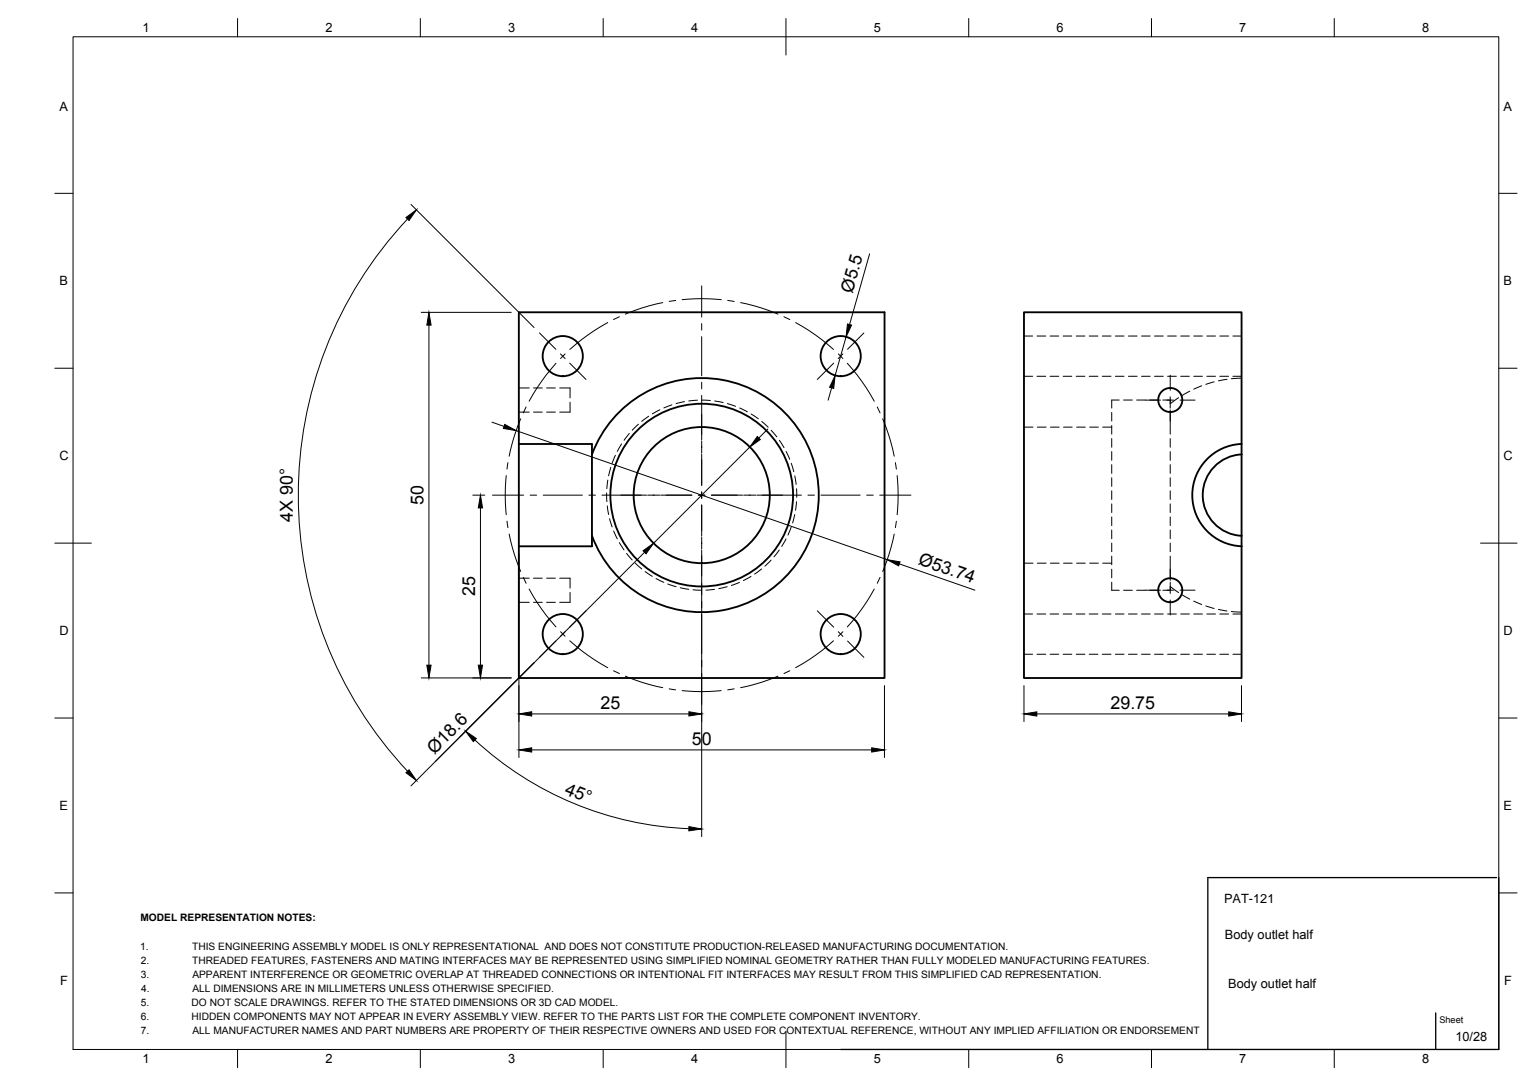
ISO-10303-21;
HEADER;
/* Generated by software containing ST-Developer
 * from STEP Tools, Inc. (www.steptools.com) 
 */

FILE_DESCRIPTION(
/* description */ ('Wall-mounted air drop station'),
/* implementation_level */ '2;1');

FILE_NAME(
/* name */ 'Body outlet half.step',
/* time_stamp */ '2026-10-28T22:16:19-07:00',
/* author */ (''),
/* organization */ (''),
/* preprocessor_version */ 'ST-DEVELOPER v20.2',
/* originating_system */ 'Autodesk Translation Framework v15.17.0.0',
/* authorisation */ '');

FILE_SCHEMA (('AUTOMOTIVE_DESIGN { 1 0 10303 214 3 1 1 }'));
ENDSEC;

DATA;
#10=MECHANICAL_DESIGN_GEOMETRIC_PRESENTATION_REPRESENTATION('',(#350),#10517);
#259=SPHERICAL_SURFACE('',#6460,1.6);
#292=SHAPE_REPRESENTATION_RELATIONSHIP('SRR','None',#10649,#321);
#321=ADVANCED_BREP_SHAPE_REPRESENTATION('',(#379),#10493);
#350=STYLED_ITEM('',(#10853),#379);
#379=MANIFOLD_SOLID_BREP('Body1',#5889);
#449=FACE_BOUND('',#1275,.T.);
#450=FACE_BOUND('',#1276,.T.);
#451=FACE_BOUND('',#1280,.T.);
#452=FACE_BOUND('',#1282,.T.);
#453=FACE_BOUND('',#1284,.T.);
#454=FACE_BOUND('',#1286,.T.);
#455=FACE_BOUND('',#1287,.T.);
#456=FACE_BOUND('',#1288,.T.);
#457=FACE_BOUND('',#1289,.T.);
#458=FACE_BOUND('',#1290,.T.);
#459=FACE_BOUND('',#1293,.T.);
#460=FACE_BOUND('',#1294,.T.);
#461=FACE_BOUND('',#1295,.T.);
#462=FACE_BOUND('',#1296,.T.);
#591=PLANE('',#6428);
#592=PLANE('',#6432);
#593=PLANE('',#6448);
#594=PLANE('',#6450);
#595=PLANE('',#6457);
#596=PLANE('',#6458);
#597=PLANE('',#6462);
#598=PLANE('',#6463);
#599=PLANE('',#6464);
#600=PLANE('',#6465);
#601=PLANE('',#6466);
#859=FACE_OUTER_BOUND('',#1264,.T.);
#860=FACE_OUTER_BOUND('',#1265,.T.);
#861=FACE_OUTER_BOUND('',#1266,.T.);
#862=FACE_OUTER_BOUND('',#1267,.T.);
#863=FACE_OUTER_BOUND('',#1268,.T.);
#864=FACE_OUTER_BOUND('',#1269,.T.);
#865=FACE_OUTER_BOUND('',#1270,.T.);
#866=FACE_OUTER_BOUND('',#1271,.T.);
#867=FACE_OUTER_BOUND('',#1272,.T.);
#868=FACE_OUTER_BOUND('',#1273,.T.);
#869=FACE_OUTER_BOUND('',#1274,.T.);
#870=FACE_OUTER_BOUND('',#1277,.T.);
#871=FACE_OUTER_BOUND('',#1278,.T.);
#872=FACE_OUTER_BOUND('',#1279,.T.);
#873=FACE_OUTER_BOUND('',#1281,.T.);
#874=FACE_OUTER_BOUND('',#1283,.T.);
#875=FACE_OUTER_BOUND('',#1285,.T.);
#876=FACE_OUTER_BOUND('',#1291,.T.);
#877=FACE_OUTER_BOUND('',#1292,.T.);
#878=FACE_OUTER_BOUND('',#1297,.T.);
#879=FACE_OUTER_BOUND('',#1298,.T.);
#1264=EDGE_LOOP('',(#4415,#4416,#4417,#4418));
#1265=EDGE_LOOP('',(#4419));
#1266=EDGE_LOOP('',(#4420,#4421,#4422,#4423));
#1267=EDGE_LOOP('',(#4424));
#1268=EDGE_LOOP('',(#4425,#4426,#4427,#4428));
#1269=EDGE_LOOP('',(#4429,#4430,#4431,#4432));
#1270=EDGE_LOOP('',(#4433,#4434,#4435,#4436));
#1271=EDGE_LOOP('',(#4437,#4438,#4439,#4440));
#1272=EDGE_LOOP('',(#4441,#4442,#4443,#4444));
#1273=EDGE_LOOP('',(#4445,#4446,#4447,#4448));
#1274=EDGE_LOOP('',(#4449,#4450,#4451,#4452,#4453,#4454));
#1275=EDGE_LOOP('',(#4455));
#1276=EDGE_LOOP('',(#4456));
#1277=EDGE_LOOP('',(#4457,#4458,#4459,#4460));
#1278=EDGE_LOOP('',(#4461,#4462,#4463,#4464));
#1279=EDGE_LOOP('',(#4465));
#1280=EDGE_LOOP('',(#4466));
#1281=EDGE_LOOP('',(#4467));
#1282=EDGE_LOOP('',(#4468));
#1283=EDGE_LOOP('',(#4469,#4470));
#1284=EDGE_LOOP('',(#4471));
#1285=EDGE_LOOP('',(#4472,#4473,#4474,#4475));
#1286=EDGE_LOOP('',(#4476));
#1287=EDGE_LOOP('',(#4477));
#1288=EDGE_LOOP('',(#4478));
#1289=EDGE_LOOP('',(#4479));
#1290=EDGE_LOOP('',(#4480));
#1291=EDGE_LOOP('',(#4481,#4482,#4483,#4484));
#1292=EDGE_LOOP('',(#4485,#4486,#4487,#4488,#4489,#4490,#4491,#4492,#4493,
#4494));
#1293=EDGE_LOOP('',(#4495));
#1294=EDGE_LOOP('',(#4496));
#1295=EDGE_LOOP('',(#4497));
#1296=EDGE_LOOP('',(#4498));
#1297=EDGE_LOOP('',(#4499,#4500,#4501,#4502));
#1298=EDGE_LOOP('',(#4503,#4504,#4505,#4506));
#1736=LINE('',#9251,#2200);
#1737=LINE('',#9258,#2201);
#1738=LINE('',#9265,#2202);
#1739=LINE('',#9271,#2203);
#1740=LINE('',#9277,#2204);
#1741=LINE('',#9283,#2205);
#1742=LINE('',#9288,#2206);
#1743=LINE('',#9292,#2207);
#1744=LINE('',#9296,#2208);
#1745=LINE('',#9299,#2209);
#1746=LINE('',#9302,#2210);
#1747=LINE('',#9304,#2211);
#1748=LINE('',#9306,#2212);
#1749=LINE('',#9308,#2213);
#1750=LINE('',#9309,#2214);
#1751=LINE('',#9314,#2215);
#1752=LINE('',#9320,#2216);
#1753=LINE('',#9331,#2217);
#1754=LINE('',#9332,#2218);
#1755=LINE('',#9333,#2219);
#1756=LINE('',#9336,#2220);
#1757=LINE('',#9337,#2221);
#1758=LINE('',#9340,#2222);
#1759=LINE('',#9341,#2223);
#1760=LINE('',#9343,#2224);
#2200=VECTOR('',#7452,0.165);
#2201=VECTOR('',#7461,0.165);
#2202=VECTOR('',#7470,0.275);
#2203=VECTOR('',#7477,0.275);
#2204=VECTOR('',#7484,0.275);
#2205=VECTOR('',#7491,0.275);
#2206=VECTOR('',#7496,1.);
#2207=VECTOR('',#7499,1.);
#2208=VECTOR('',#7504,1.);
#2209=VECTOR('',#7507,1.);
#2210=VECTOR('',#7510,1.);
#2211=VECTOR('',#7511,1.);
#2212=VECTOR('',#7512,1.);
#2213=VECTOR('',#7513,1.);
#2214=VECTOR('',#7514,1.);
#2215=VECTOR('',#7519,0.93);
#2216=VECTOR('',#7526,1.3);
#2217=VECTOR('',#7541,1.);
#2218=VECTOR('',#7542,1.);
#2219=VECTOR('',#7543,1.);
#2220=VECTOR('',#7546,1.);
#2221=VECTOR('',#7547,1.);
#2222=VECTOR('',#7550,1.);
#2223=VECTOR('',#7551,1.);
#2224=VECTOR('',#7554,1.);
#2597=CIRCLE('',#6426,0.165);
#2598=CIRCLE('',#6427,0.165);
#2599=CIRCLE('',#6430,0.165);
#2600=CIRCLE('',#6431,0.165);
#2601=CIRCLE('',#6434,0.275);
#2602=CIRCLE('',#6435,0.275);
#2603=CIRCLE('',#6437,0.275);
#2604=CIRCLE('',#6438,0.275);
#2605=CIRCLE('',#6440,0.275);
#2606=CIRCLE('',#6441,0.275);
#2607=CIRCLE('',#6443,0.275);
#2608=CIRCLE('',#6444,0.275);
#2609=CIRCLE('',#6446,0.7);
#2610=CIRCLE('',#6447,0.7);
#2611=CIRCLE('',#6449,0.556776436283003);
#2612=CIRCLE('',#6452,0.93);
#2613=CIRCLE('',#6453,0.93);
#2614=CIRCLE('',#6455,1.3);
#2615=CIRCLE('',#6456,1.3);
#2616=CIRCLE('',#6459,1.24899959967968);
#2617=CIRCLE('',#6461,1.59980467557762);
#2912=VERTEX_POINT('',#9248);
#2913=VERTEX_POINT('',#9250);
#2914=VERTEX_POINT('',#9255);
#2915=VERTEX_POINT('',#9257);
#2916=VERTEX_POINT('',#9262);
#2917=VERTEX_POINT('',#9264);
#2918=VERTEX_POINT('',#9268);
#2919=VERTEX_POINT('',#9270);
#2920=VERTEX_POINT('',#9274);
#2921=VERTEX_POINT('',#9276);
#2922=VERTEX_POINT('',#9280);
#2923=VERTEX_POINT('',#9282);
#2924=VERTEX_POINT('',#9286);
#2925=VERTEX_POINT('',#9287);
#2926=VERTEX_POINT('',#9289);
#2927=VERTEX_POINT('',#9291);
#2928=VERTEX_POINT('',#9295);
#2929=VERTEX_POINT('',#9297);
#2930=VERTEX_POINT('',#9301);
#2931=VERTEX_POINT('',#9303);
#2932=VERTEX_POINT('',#9305);
#2933=VERTEX_POINT('',#9307);
#2934=VERTEX_POINT('',#9311);
#2935=VERTEX_POINT('',#9313);
#2936=VERTEX_POINT('',#9317);
#2937=VERTEX_POINT('',#9319);
#2938=VERTEX_POINT('',#9324);
#2939=VERTEX_POINT('',#9329);
#2940=VERTEX_POINT('',#9330);
#2941=VERTEX_POINT('',#9335);
#2942=VERTEX_POINT('',#9339);
#3465=EDGE_CURVE('',#2912,#2912,#2597,.T.);
#3466=EDGE_CURVE('',#2912,#2913,#1736,.T.);
#3467=EDGE_CURVE('',#2913,#2913,#2598,.T.);
#3468=EDGE_CURVE('',#2914,#2914,#2599,.T.);
#3469=EDGE_CURVE('',#2914,#2915,#1737,.T.);
#3470=EDGE_CURVE('',#2915,#2915,#2600,.T.);
#3471=EDGE_CURVE('',#2916,#2916,#2601,.T.);
#3472=EDGE_CURVE('',#2916,#2917,#1738,.T.);
#3473=EDGE_CURVE('',#2917,#2917,#2602,.T.);
#3474=EDGE_CURVE('',#2918,#2918,#2603,.T.);
#3475=EDGE_CURVE('',#2918,#2919,#1739,.T.);
#3476=EDGE_CURVE('',#2919,#2919,#2604,.T.);
#3477=EDGE_CURVE('',#2920,#2920,#2605,.T.);
#3478=EDGE_CURVE('',#2920,#2921,#1740,.T.);
#3479=EDGE_CURVE('',#2921,#2921,#2606,.T.);
#3480=EDGE_CURVE('',#2922,#2922,#2607,.T.);
#3481=EDGE_CURVE('',#2922,#2923,#1741,.T.);
#3482=EDGE_CURVE('',#2923,#2923,#2608,.T.);
#3483=EDGE_CURVE('',#2924,#2925,#1742,.T.);
#3484=EDGE_CURVE('',#2926,#2924,#2609,.T.);
#3485=EDGE_CURVE('',#2927,#2926,#1743,.T.);
#3486=EDGE_CURVE('',#2925,#2927,#2610,.T.);
#3487=EDGE_CURVE('',#2928,#2924,#1744,.T.);
#3488=EDGE_CURVE('',#2929,#2928,#2611,.T.);
#3489=EDGE_CURVE('',#2926,#2929,#1745,.T.);
#3490=EDGE_CURVE('',#2927,#2930,#1746,.T.);
#3491=EDGE_CURVE('',#2930,#2931,#1747,.T.);
#3492=EDGE_CURVE('',#2931,#2932,#1748,.T.);
#3493=EDGE_CURVE('',#2932,#2933,#1749,.T.);
#3494=EDGE_CURVE('',#2933,#2925,#1750,.T.);
#3495=EDGE_CURVE('',#2934,#2934,#2612,.T.);
#3496=EDGE_CURVE('',#2934,#2935,#1751,.T.);
#3497=EDGE_CURVE('',#2935,#2935,#2613,.T.);
#3498=EDGE_CURVE('',#2936,#2936,#2614,.T.);
#3499=EDGE_CURVE('',#2936,#2937,#1752,.T.);
#3500=EDGE_CURVE('',#2937,#2937,#2615,.T.);
#3501=EDGE_CURVE('',#2938,#2938,#2616,.T.);
#3502=EDGE_CURVE('',#2929,#2928,#2617,.T.);
#3503=EDGE_CURVE('',#2939,#2940,#1753,.T.);
#3504=EDGE_CURVE('',#2940,#2932,#1754,.T.);
#3505=EDGE_CURVE('',#2939,#2931,#1755,.T.);
#3506=EDGE_CURVE('',#2941,#2939,#1756,.T.);
#3507=EDGE_CURVE('',#2941,#2930,#1757,.T.);
#3508=EDGE_CURVE('',#2942,#2933,#1758,.T.);
#3509=EDGE_CURVE('',#2942,#2941,#1759,.T.);
#3510=EDGE_CURVE('',#2940,#2942,#1760,.T.);
#4415=ORIENTED_EDGE('',*,*,#3465,.F.);
#4416=ORIENTED_EDGE('',*,*,#3466,.T.);
#4417=ORIENTED_EDGE('',*,*,#3467,.F.);
#4418=ORIENTED_EDGE('',*,*,#3466,.F.);
#4419=ORIENTED_EDGE('',*,*,#3465,.T.);
#4420=ORIENTED_EDGE('',*,*,#3468,.F.);
#4421=ORIENTED_EDGE('',*,*,#3469,.T.);
#4422=ORIENTED_EDGE('',*,*,#3470,.F.);
#4423=ORIENTED_EDGE('',*,*,#3469,.F.);
#4424=ORIENTED_EDGE('',*,*,#3468,.T.);
#4425=ORIENTED_EDGE('',*,*,#3471,.F.);
#4426=ORIENTED_EDGE('',*,*,#3472,.T.);
#4427=ORIENTED_EDGE('',*,*,#3473,.F.);
#4428=ORIENTED_EDGE('',*,*,#3472,.F.);
#4429=ORIENTED_EDGE('',*,*,#3474,.F.);
#4430=ORIENTED_EDGE('',*,*,#3475,.T.);
#4431=ORIENTED_EDGE('',*,*,#3476,.F.);
#4432=ORIENTED_EDGE('',*,*,#3475,.F.);
#4433=ORIENTED_EDGE('',*,*,#3477,.F.);
#4434=ORIENTED_EDGE('',*,*,#3478,.T.);
#4435=ORIENTED_EDGE('',*,*,#3479,.F.);
#4436=ORIENTED_EDGE('',*,*,#3478,.F.);
#4437=ORIENTED_EDGE('',*,*,#3480,.F.);
#4438=ORIENTED_EDGE('',*,*,#3481,.T.);
#4439=ORIENTED_EDGE('',*,*,#3482,.F.);
#4440=ORIENTED_EDGE('',*,*,#3481,.F.);
#4441=ORIENTED_EDGE('',*,*,#3483,.F.);
#4442=ORIENTED_EDGE('',*,*,#3484,.F.);
#4443=ORIENTED_EDGE('',*,*,#3485,.F.);
#4444=ORIENTED_EDGE('',*,*,#3486,.F.);
#4445=ORIENTED_EDGE('',*,*,#3487,.F.);
#4446=ORIENTED_EDGE('',*,*,#3488,.F.);
#4447=ORIENTED_EDGE('',*,*,#3489,.F.);
#4448=ORIENTED_EDGE('',*,*,#3484,.T.);
#4449=ORIENTED_EDGE('',*,*,#3486,.T.);
#4450=ORIENTED_EDGE('',*,*,#3490,.T.);
#4451=ORIENTED_EDGE('',*,*,#3491,.T.);
#4452=ORIENTED_EDGE('',*,*,#3492,.T.);
#4453=ORIENTED_EDGE('',*,*,#3493,.T.);
#4454=ORIENTED_EDGE('',*,*,#3494,.T.);
#4455=ORIENTED_EDGE('',*,*,#3467,.T.);
#4456=ORIENTED_EDGE('',*,*,#3470,.T.);
#4457=ORIENTED_EDGE('',*,*,#3495,.F.);
#4458=ORIENTED_EDGE('',*,*,#3496,.T.);
#4459=ORIENTED_EDGE('',*,*,#3497,.F.);
#4460=ORIENTED_EDGE('',*,*,#3496,.F.);
#4461=ORIENTED_EDGE('',*,*,#3498,.F.);
#4462=ORIENTED_EDGE('',*,*,#3499,.T.);
#4463=ORIENTED_EDGE('',*,*,#3500,.T.);
#4464=ORIENTED_EDGE('',*,*,#3499,.F.);
#4465=ORIENTED_EDGE('',*,*,#3500,.F.);
#4466=ORIENTED_EDGE('',*,*,#3495,.T.);
#4467=ORIENTED_EDGE('',*,*,#3498,.T.);
#4468=ORIENTED_EDGE('',*,*,#3501,.F.);
#4469=ORIENTED_EDGE('',*,*,#3488,.T.);
#4470=ORIENTED_EDGE('',*,*,#3502,.F.);
#4471=ORIENTED_EDGE('',*,*,#3501,.T.);
#4472=ORIENTED_EDGE('',*,*,#3503,.T.);
#4473=ORIENTED_EDGE('',*,*,#3504,.T.);
#4474=ORIENTED_EDGE('',*,*,#3492,.F.);
#4475=ORIENTED_EDGE('',*,*,#3505,.F.);
#4476=ORIENTED_EDGE('',*,*,#3497,.T.);
#4477=ORIENTED_EDGE('',*,*,#3482,.T.);
#4478=ORIENTED_EDGE('',*,*,#3479,.T.);
#4479=ORIENTED_EDGE('',*,*,#3476,.T.);
#4480=ORIENTED_EDGE('',*,*,#3473,.T.);
#4481=ORIENTED_EDGE('',*,*,#3506,.T.);
#4482=ORIENTED_EDGE('',*,*,#3505,.T.);
#4483=ORIENTED_EDGE('',*,*,#3491,.F.);
#4484=ORIENTED_EDGE('',*,*,#3507,.F.);
#4485=ORIENTED_EDGE('',*,*,#3483,.T.);
#4486=ORIENTED_EDGE('',*,*,#3494,.F.);
#4487=ORIENTED_EDGE('',*,*,#3508,.F.);
#4488=ORIENTED_EDGE('',*,*,#3509,.T.);
#4489=ORIENTED_EDGE('',*,*,#3507,.T.);
#4490=ORIENTED_EDGE('',*,*,#3490,.F.);
#4491=ORIENTED_EDGE('',*,*,#3485,.T.);
#4492=ORIENTED_EDGE('',*,*,#3489,.T.);
#4493=ORIENTED_EDGE('',*,*,#3502,.T.);
#4494=ORIENTED_EDGE('',*,*,#3487,.T.);
#4495=ORIENTED_EDGE('',*,*,#3471,.T.);
#4496=ORIENTED_EDGE('',*,*,#3474,.T.);
#4497=ORIENTED_EDGE('',*,*,#3477,.T.);
#4498=ORIENTED_EDGE('',*,*,#3480,.T.);
#4499=ORIENTED_EDGE('',*,*,#3510,.T.);
#4500=ORIENTED_EDGE('',*,*,#3508,.T.);
#4501=ORIENTED_EDGE('',*,*,#3493,.F.);
#4502=ORIENTED_EDGE('',*,*,#3504,.F.);
#4503=ORIENTED_EDGE('',*,*,#3510,.F.);
#4504=ORIENTED_EDGE('',*,*,#3503,.F.);
#4505=ORIENTED_EDGE('',*,*,#3506,.F.);
#4506=ORIENTED_EDGE('',*,*,#3509,.F.);
#5466=CYLINDRICAL_SURFACE('',#6425,0.165);
#5467=CYLINDRICAL_SURFACE('',#6429,0.165);
#5468=CYLINDRICAL_SURFACE('',#6433,0.275);
#5469=CYLINDRICAL_SURFACE('',#6436,0.275);
#5470=CYLINDRICAL_SURFACE('',#6439,0.275);
#5471=CYLINDRICAL_SURFACE('',#6442,0.275);
#5472=CYLINDRICAL_SURFACE('',#6445,0.7);
#5473=CYLINDRICAL_SURFACE('',#6451,0.93);
#5474=CYLINDRICAL_SURFACE('',#6454,1.3);
#5632=ADVANCED_FACE('',(#859),#5466,.F.);
#5633=ADVANCED_FACE('',(#860),#591,.T.);
#5634=ADVANCED_FACE('',(#861),#5467,.F.);
#5635=ADVANCED_FACE('',(#862),#592,.T.);
#5636=ADVANCED_FACE('',(#863),#5468,.F.);
#5637=ADVANCED_FACE('',(#864),#5469,.F.);
#5638=ADVANCED_FACE('',(#865),#5470,.F.);
#5639=ADVANCED_FACE('',(#866),#5471,.F.);
#5640=ADVANCED_FACE('',(#867),#5472,.F.);
#5641=ADVANCED_FACE('',(#868),#593,.T.);
#5642=ADVANCED_FACE('',(#869,#449,#450),#594,.T.);
#5643=ADVANCED_FACE('',(#870),#5473,.F.);
#5644=ADVANCED_FACE('',(#871),#5474,.F.);
#5645=ADVANCED_FACE('',(#872,#451),#595,.F.);
#5646=ADVANCED_FACE('',(#873,#452),#596,.T.);
#5647=ADVANCED_FACE('',(#874,#453),#259,.F.);
#5648=ADVANCED_FACE('',(#875,#454,#455,#456,#457,#458),#597,.T.);
#5649=ADVANCED_FACE('',(#876),#598,.T.);
#5650=ADVANCED_FACE('',(#877,#459,#460,#461,#462),#599,.T.);
#5651=ADVANCED_FACE('',(#878),#600,.T.);
#5652=ADVANCED_FACE('',(#879),#601,.F.);
#5889=CLOSED_SHELL('',(#5632,#5633,#5634,#5635,#5636,#5637,#5638,#5639,
#5640,#5641,#5642,#5643,#5644,#5645,#5646,#5647,#5648,#5649,#5650,#5651,
#5652));
#6424=AXIS2_PLACEMENT_3D('',#9246,#7446,#7447);
#6425=AXIS2_PLACEMENT_3D('',#9247,#7448,#7449);
#6426=AXIS2_PLACEMENT_3D('',#9249,#7450,#7451);
#6427=AXIS2_PLACEMENT_3D('',#9252,#7453,#7454);
#6428=AXIS2_PLACEMENT_3D('',#9253,#7455,#7456);
#6429=AXIS2_PLACEMENT_3D('',#9254,#7457,#7458);
#6430=AXIS2_PLACEMENT_3D('',#9256,#7459,#7460);
#6431=AXIS2_PLACEMENT_3D('',#9259,#7462,#7463);
#6432=AXIS2_PLACEMENT_3D('',#9260,#7464,#7465);
#6433=AXIS2_PLACEMENT_3D('',#9261,#7466,#7467);
#6434=AXIS2_PLACEMENT_3D('',#9263,#7468,#7469);
#6435=AXIS2_PLACEMENT_3D('',#9266,#7471,#7472);
#6436=AXIS2_PLACEMENT_3D('',#9267,#7473,#7474);
#6437=AXIS2_PLACEMENT_3D('',#9269,#7475,#7476);
#6438=AXIS2_PLACEMENT_3D('',#9272,#7478,#7479);
#6439=AXIS2_PLACEMENT_3D('',#9273,#7480,#7481);
#6440=AXIS2_PLACEMENT_3D('',#9275,#7482,#7483);
#6441=AXIS2_PLACEMENT_3D('',#9278,#7485,#7486);
#6442=AXIS2_PLACEMENT_3D('',#9279,#7487,#7488);
#6443=AXIS2_PLACEMENT_3D('',#9281,#7489,#7490);
#6444=AXIS2_PLACEMENT_3D('',#9284,#7492,#7493);
#6445=AXIS2_PLACEMENT_3D('',#9285,#7494,#7495);
#6446=AXIS2_PLACEMENT_3D('',#9290,#7497,#7498);
#6447=AXIS2_PLACEMENT_3D('',#9293,#7500,#7501);
#6448=AXIS2_PLACEMENT_3D('',#9294,#7502,#7503);
#6449=AXIS2_PLACEMENT_3D('',#9298,#7505,#7506);
#6450=AXIS2_PLACEMENT_3D('',#9300,#7508,#7509);
#6451=AXIS2_PLACEMENT_3D('',#9310,#7515,#7516);
#6452=AXIS2_PLACEMENT_3D('',#9312,#7517,#7518);
#6453=AXIS2_PLACEMENT_3D('',#9315,#7520,#7521);
#6454=AXIS2_PLACEMENT_3D('',#9316,#7522,#7523);
#6455=AXIS2_PLACEMENT_3D('',#9318,#7524,#7525);
#6456=AXIS2_PLACEMENT_3D('',#9321,#7527,#7528);
#6457=AXIS2_PLACEMENT_3D('',#9322,#7529,#7530);
#6458=AXIS2_PLACEMENT_3D('',#9323,#7531,#7532);
#6459=AXIS2_PLACEMENT_3D('',#9325,#7533,#7534);
#6460=AXIS2_PLACEMENT_3D('',#9326,#7535,#7536);
#6461=AXIS2_PLACEMENT_3D('',#9327,#7537,#7538);
#6462=AXIS2_PLACEMENT_3D('',#9328,#7539,#7540);
#6463=AXIS2_PLACEMENT_3D('',#9334,#7544,#7545);
#6464=AXIS2_PLACEMENT_3D('',#9338,#7548,#7549);
#6465=AXIS2_PLACEMENT_3D('',#9342,#7552,#7553);
#6466=AXIS2_PLACEMENT_3D('',#9344,#7555,#7556);
#7446=DIRECTION('axis',(0.,0.,1.));
#7447=DIRECTION('refdir',(1.,0.,0.));
#7448=DIRECTION('center_axis',(0.,0.,1.));
#7449=DIRECTION('ref_axis',(1.,0.,0.));
#7450=DIRECTION('center_axis',(0.,0.,1.));
#7451=DIRECTION('ref_axis',(1.,0.,0.));
#7452=DIRECTION('',(0.,0.,1.));
#7453=DIRECTION('center_axis',(0.,0.,-1.));
#7454=DIRECTION('ref_axis',(1.,0.,0.));
#7455=DIRECTION('center_axis',(0.,0.,1.));
#7456=DIRECTION('ref_axis',(1.,0.,0.));
#7457=DIRECTION('center_axis',(0.,0.,1.));
#7458=DIRECTION('ref_axis',(1.,0.,0.));
#7459=DIRECTION('center_axis',(0.,0.,1.));
#7460=DIRECTION('ref_axis',(1.,0.,0.));
#7461=DIRECTION('',(0.,0.,1.));
#7462=DIRECTION('center_axis',(0.,0.,-1.));
#7463=DIRECTION('ref_axis',(1.,0.,0.));
#7464=DIRECTION('center_axis',(0.,0.,1.));
#7465=DIRECTION('ref_axis',(1.,0.,0.));
#7466=DIRECTION('center_axis',(0.,1.,0.));
#7467=DIRECTION('ref_axis',(1.,0.,0.));
#7468=DIRECTION('center_axis',(0.,1.,0.));
#7469=DIRECTION('ref_axis',(1.,0.,0.));
#7470=DIRECTION('',(0.,1.,0.));
#7471=DIRECTION('center_axis',(0.,-1.,0.));
#7472=DIRECTION('ref_axis',(1.,0.,0.));
#7473=DIRECTION('center_axis',(0.,1.,0.));
#7474=DIRECTION('ref_axis',(1.,0.,0.));
#7475=DIRECTION('center_axis',(0.,1.,0.));
#7476=DIRECTION('ref_axis',(1.,0.,0.));
#7477=DIRECTION('',(0.,1.,0.));
#7478=DIRECTION('center_axis',(0.,-1.,0.));
#7479=DIRECTION('ref_axis',(1.,0.,0.));
#7480=DIRECTION('center_axis',(0.,1.,0.));
#7481=DIRECTION('ref_axis',(1.,0.,0.));
#7482=DIRECTION('center_axis',(0.,1.,0.));
#7483=DIRECTION('ref_axis',(1.,0.,0.));
#7484=DIRECTION('',(0.,1.,0.));
#7485=DIRECTION('center_axis',(0.,-1.,0.));
#7486=DIRECTION('ref_axis',(1.,0.,0.));
#7487=DIRECTION('center_axis',(0.,1.,0.));
#7488=DIRECTION('ref_axis',(1.,0.,0.));
#7489=DIRECTION('center_axis',(0.,1.,0.));
#7490=DIRECTION('ref_axis',(1.,0.,0.));
#7491=DIRECTION('',(0.,1.,0.));
#7492=DIRECTION('center_axis',(0.,-1.,0.));
#7493=DIRECTION('ref_axis',(1.,0.,0.));
#7494=DIRECTION('center_axis',(0.,0.,1.));
#7495=DIRECTION('ref_axis',(1.,0.,0.));
#7496=DIRECTION('',(0.,0.,1.));
#7497=DIRECTION('center_axis',(0.,0.,1.));
#7498=DIRECTION('ref_axis',(1.,0.,0.));
#7499=DIRECTION('',(0.,0.,-1.));
#7500=DIRECTION('center_axis',(0.,0.,-1.));
#7501=DIRECTION('ref_axis',(1.,0.,0.));
#7502=DIRECTION('center_axis',(0.,0.,1.));
#7503=DIRECTION('ref_axis',(1.,0.,0.));
#7504=DIRECTION('',(-1.,0.,0.));
#7505=DIRECTION('center_axis',(0.,0.,1.));
#7506=DIRECTION('ref_axis',(0.,-1.,0.));
#7507=DIRECTION('',(-1.,0.,0.));
#7508=DIRECTION('center_axis',(0.,0.,1.));
#7509=DIRECTION('ref_axis',(1.,0.,0.));
#7510=DIRECTION('',(1.,0.,0.));
#7511=DIRECTION('',(0.,1.,0.));
#7512=DIRECTION('',(-1.,0.,0.));
#7513=DIRECTION('',(0.,-1.,0.));
#7514=DIRECTION('',(1.,0.,0.));
#7515=DIRECTION('center_axis',(0.,1.,0.));
#7516=DIRECTION('ref_axis',(1.,0.,0.));
#7517=DIRECTION('center_axis',(0.,1.,0.));
#7518=DIRECTION('ref_axis',(1.,0.,0.));
#7519=DIRECTION('',(0.,1.,0.));
#7520=DIRECTION('center_axis',(0.,-1.,0.));
#7521=DIRECTION('ref_axis',(1.,0.,0.));
#7522=DIRECTION('center_axis',(0.,1.,0.));
#7523=DIRECTION('ref_axis',(1.,0.,0.));
#7524=DIRECTION('center_axis',(0.,1.,0.));
#7525=DIRECTION('ref_axis',(1.,0.,0.));
#7526=DIRECTION('',(0.,1.,0.));
#7527=DIRECTION('center_axis',(0.,1.,0.));
#7528=DIRECTION('ref_axis',(1.,0.,0.));
#7529=DIRECTION('center_axis',(0.,1.,0.));
#7530=DIRECTION('ref_axis',(1.,0.,0.));
#7531=DIRECTION('center_axis',(0.,1.,0.));
#7532=DIRECTION('ref_axis',(1.,0.,0.));
#7533=DIRECTION('center_axis',(0.,1.,0.));
#7534=DIRECTION('ref_axis',(0.,0.,1.));
#7535=DIRECTION('center_axis',(6.12323399573677E-17,0.,1.));
#7536=DIRECTION('ref_axis',(1.,0.,0.));
#7537=DIRECTION('center_axis',(0.,1.,0.));
#7538=DIRECTION('ref_axis',(0.,0.,1.));
#7539=DIRECTION('center_axis',(0.,1.,0.));
#7540=DIRECTION('ref_axis',(-1.,0.,0.));
#7541=DIRECTION('',(-1.,0.,0.));
#7542=DIRECTION('',(0.,0.,1.));
#7543=DIRECTION('',(0.,0.,1.));
#7544=DIRECTION('center_axis',(1.,0.,0.));
#7545=DIRECTION('ref_axis',(0.,1.,0.));
#7546=DIRECTION('',(0.,1.,0.));
#7547=DIRECTION('',(0.,0.,1.));
#7548=DIRECTION('center_axis',(0.,-1.,0.));
#7549=DIRECTION('ref_axis',(1.,0.,0.));
#7550=DIRECTION('',(0.,0.,1.));
#7551=DIRECTION('',(1.,0.,0.));
#7552=DIRECTION('center_axis',(-1.,0.,0.));
#7553=DIRECTION('ref_axis',(0.,-1.,0.));
#7554=DIRECTION('',(0.,-1.,0.));
#7555=DIRECTION('center_axis',(0.,0.,1.));
#7556=DIRECTION('ref_axis',(1.,0.,0.));
#9246=CARTESIAN_POINT('',(0.,0.,0.));
#9247=CARTESIAN_POINT('Origin',(-1.3,1.,6.8));
#9248=CARTESIAN_POINT('',(-1.465,1.,6.8));
#9249=CARTESIAN_POINT('Origin',(-1.3,1.,6.8));
#9250=CARTESIAN_POINT('',(-1.465,1.,7.5));
#9251=CARTESIAN_POINT('',(-1.465,1.,6.8));
#9252=CARTESIAN_POINT('Origin',(-1.3,1.,7.5));
#9253=CARTESIAN_POINT('Origin',(-1.3,1.,6.8));
#9254=CARTESIAN_POINT('Origin',(1.3,1.,6.8));
#9255=CARTESIAN_POINT('',(1.135,1.,6.8));
#9256=CARTESIAN_POINT('Origin',(1.3,1.,6.8));
#9257=CARTESIAN_POINT('',(1.135,1.,7.5));
#9258=CARTESIAN_POINT('',(1.135,1.,6.8));
#9259=CARTESIAN_POINT('Origin',(1.3,1.,7.5));
#9260=CARTESIAN_POINT('Origin',(1.3,1.,6.8));
#9261=CARTESIAN_POINT('Origin',(1.9,-3.1,3.1));
#9262=CARTESIAN_POINT('',(1.625,0.0249999999999999,3.1));
#9263=CARTESIAN_POINT('Origin',(1.9,0.0249999999999999,3.1));
#9264=CARTESIAN_POINT('',(1.625,3.,3.1));
#9265=CARTESIAN_POINT('',(1.625,-3.1,3.1));
#9266=CARTESIAN_POINT('Origin',(1.9,3.,3.1));
#9267=CARTESIAN_POINT('Origin',(-1.9,-3.1,6.9));
#9268=CARTESIAN_POINT('',(-2.175,0.0249999999999999,6.9));
#9269=CARTESIAN_POINT('Origin',(-1.9,0.0249999999999999,6.9));
#9270=CARTESIAN_POINT('',(-2.175,3.,6.9));
#9271=CARTESIAN_POINT('',(-2.175,-3.1,6.9));
#9272=CARTESIAN_POINT('Origin',(-1.9,3.,6.9));
#9273=CARTESIAN_POINT('Origin',(-1.9,-3.1,3.1));
#9274=CARTESIAN_POINT('',(-2.175,0.0249999999999999,3.1));
#9275=CARTESIAN_POINT('Origin',(-1.9,0.0249999999999999,3.1));
#9276=CARTESIAN_POINT('',(-2.175,3.,3.1));
#9277=CARTESIAN_POINT('',(-2.175,-3.1,3.1));
#9278=CARTESIAN_POINT('Origin',(-1.9,3.,3.1));
#9279=CARTESIAN_POINT('Origin',(1.9,-3.1,6.9));
#9280=CARTESIAN_POINT('',(1.625,0.0249999999999999,6.9));
#9281=CARTESIAN_POINT('Origin',(1.9,0.0249999999999999,6.9));
#9282=CARTESIAN_POINT('',(1.625,3.,6.9));
#9283=CARTESIAN_POINT('',(1.625,-3.1,6.9));
#9284=CARTESIAN_POINT('Origin',(1.9,3.,6.9));
#9285=CARTESIAN_POINT('Origin',(0.,0.,6.5));
#9286=CARTESIAN_POINT('',(-0.699553428981661,0.025,6.5));
#9287=CARTESIAN_POINT('',(-0.699553428981661,0.025,7.5));
#9288=CARTESIAN_POINT('',(-0.699553428981661,0.025,6.5));
#9289=CARTESIAN_POINT('',(0.699553428981661,0.025,6.5));
#9290=CARTESIAN_POINT('Origin',(0.,0.,6.5));
#9291=CARTESIAN_POINT('',(0.699553428981661,0.025,7.5));
#9292=CARTESIAN_POINT('',(0.699553428981661,0.025,6.5));
#9293=CARTESIAN_POINT('Origin',(0.,0.,7.5));
#9294=CARTESIAN_POINT('Origin',(0.,0.,6.5));
#9295=CARTESIAN_POINT('',(-0.556214886532175,0.025,6.5));
#9296=CARTESIAN_POINT('',(-1.25,0.025,6.5));
#9297=CARTESIAN_POINT('',(0.556214886532175,0.025,6.5));
#9298=CARTESIAN_POINT('Origin',(0.,0.,6.5));
#9299=CARTESIAN_POINT('',(-1.25,0.025,6.5));
#9300=CARTESIAN_POINT('Origin',(0.,1.5125,7.5));
#9301=CARTESIAN_POINT('',(2.5,0.0249999999999999,7.5));
#9302=CARTESIAN_POINT('',(-2.5,0.025,7.5));
#9303=CARTESIAN_POINT('',(2.5,3.,7.5));
#9304=CARTESIAN_POINT('',(2.5,0.025,7.5));
#9305=CARTESIAN_POINT('',(-2.5,3.,7.5));
#9306=CARTESIAN_POINT('',(2.5,3.,7.5));
#9307=CARTESIAN_POINT('',(-2.5,0.0249999999999999,7.5));
#9308=CARTESIAN_POINT('',(-2.5,3.,7.5));
#9309=CARTESIAN_POINT('',(-2.5,0.025,7.5));
#9310=CARTESIAN_POINT('Origin',(0.,1.8,5.));
#9311=CARTESIAN_POINT('',(-0.93,1.8,5.));
#9312=CARTESIAN_POINT('Origin',(0.,1.8,5.));
#9313=CARTESIAN_POINT('',(-0.93,3.,5.));
#9314=CARTESIAN_POINT('',(-0.93,1.8,5.));
#9315=CARTESIAN_POINT('Origin',(0.,3.,5.));
#9316=CARTESIAN_POINT('Origin',(0.,1.,5.));
#9317=CARTESIAN_POINT('',(-1.3,1.,5.));
#9318=CARTESIAN_POINT('Origin',(0.,1.,5.));
#9319=CARTESIAN_POINT('',(-1.3,1.8,5.));
#9320=CARTESIAN_POINT('',(-1.3,1.,5.));
#9321=CARTESIAN_POINT('Origin',(0.,1.8,5.));
#9322=CARTESIAN_POINT('Origin',(0.,1.8,5.));
#9323=CARTESIAN_POINT('Origin',(0.,1.,5.));
#9324=CARTESIAN_POINT('',(-1.52958336188405E-16,1.,3.75100040032032));
#9325=CARTESIAN_POINT('Origin',(0.,1.,5.));
#9326=CARTESIAN_POINT('Origin',(0.,0.,5.));
#9327=CARTESIAN_POINT('Origin',(0.,0.025,5.));
#9328=CARTESIAN_POINT('Origin',(2.5,3.,2.5));
#9329=CARTESIAN_POINT('',(2.5,3.,2.5));
#9330=CARTESIAN_POINT('',(-2.5,3.,2.5));
#9331=CARTESIAN_POINT('',(2.5,3.,2.5));
#9332=CARTESIAN_POINT('',(-2.5,3.,2.5));
#9333=CARTESIAN_POINT('',(2.5,3.,2.5));
#9334=CARTESIAN_POINT('Origin',(2.5,0.025,2.5));
#9335=CARTESIAN_POINT('',(2.5,0.025,2.5));
#9336=CARTESIAN_POINT('',(2.5,0.025,2.5));
#9337=CARTESIAN_POINT('',(2.5,0.025,2.5));
#9338=CARTESIAN_POINT('Origin',(-2.5,0.025,2.5));
#9339=CARTESIAN_POINT('',(-2.5,0.0249999999999999,2.5));
#9340=CARTESIAN_POINT('',(-2.5,0.0249999999999999,2.5));
#9341=CARTESIAN_POINT('',(-2.5,0.025,2.5));
#9342=CARTESIAN_POINT('Origin',(-2.5,3.,2.5));
#9343=CARTESIAN_POINT('',(-2.5,3.,2.5));
#9344=CARTESIAN_POINT('Origin',(0.,1.5125,2.5));
#10460=UNCERTAINTY_MEASURE_WITH_UNIT(LENGTH_MEASURE(0.001),#10518,
'DISTANCE_ACCURACY_VALUE',
'Maximum model space distance between geometric entities at asserted c
onnectivities');
#10484=UNCERTAINTY_MEASURE_WITH_UNIT(LENGTH_MEASURE(0.001),#10518,
'DISTANCE_ACCURACY_VALUE',
'Maximum model space distance between geometric entities at asserted c
onnectivities');
#10493=(
GEOMETRIC_REPRESENTATION_CONTEXT(3)
GLOBAL_UNCERTAINTY_ASSIGNED_CONTEXT((#10460))
GLOBAL_UNIT_ASSIGNED_CONTEXT((#10518,#10520,#10521))
REPRESENTATION_CONTEXT('','3D')
);
#10517=(
GEOMETRIC_REPRESENTATION_CONTEXT(3)
GLOBAL_UNCERTAINTY_ASSIGNED_CONTEXT((#10484))
GLOBAL_UNIT_ASSIGNED_CONTEXT((#10518,#10520,#10521))
REPRESENTATION_CONTEXT('','3D')
);
#10518=(
LENGTH_UNIT()
NAMED_UNIT(*)
SI_UNIT(.CENTI.,.METRE.)
);
#10520=(
NAMED_UNIT(*)
PLANE_ANGLE_UNIT()
SI_UNIT($,.RADIAN.)
);
#10521=(
NAMED_UNIT(*)
SI_UNIT($,.STERADIAN.)
SOLID_ANGLE_UNIT()
);
#10530=SHAPE_DEFINITION_REPRESENTATION(#10562,#10649);
#10562=PRODUCT_DEFINITION_SHAPE('',$,#10682);
#10649=SHAPE_REPRESENTATION('',(#6424),#10493);
#10673=PRODUCT_DEFINITION_CONTEXT('part definition',#10771,'design');
#10682=PRODUCT_DEFINITION('Body outlet half','Body outlet half',#10714,
#10673);
#10714=PRODUCT_DEFINITION_FORMATION('',$,#10781);
#10771=APPLICATION_CONTEXT(
'Core Data for Automotive Mechanical Design Process');
#10772=PRODUCT_CONTEXT('part definition',#10771,'mechanical');
#10781=PRODUCT('Body outlet half','Body outlet half','Body outlet half',
(#10772));
#10847=COLOUR_RGB('Dark Blue',0.08,0.2,0.34);
#10848=FILL_AREA_STYLE_COLOUR('',#10847);
#10849=FILL_AREA_STYLE('',(#10848));
#10850=SURFACE_STYLE_FILL_AREA(#10849);
#10851=SURFACE_SIDE_STYLE('',(#10850));
#10852=SURFACE_STYLE_USAGE(.BOTH.,#10851);
#10853=PRESENTATION_STYLE_ASSIGNMENT((#10852));
ENDSEC;
END-ISO-10303-21;
